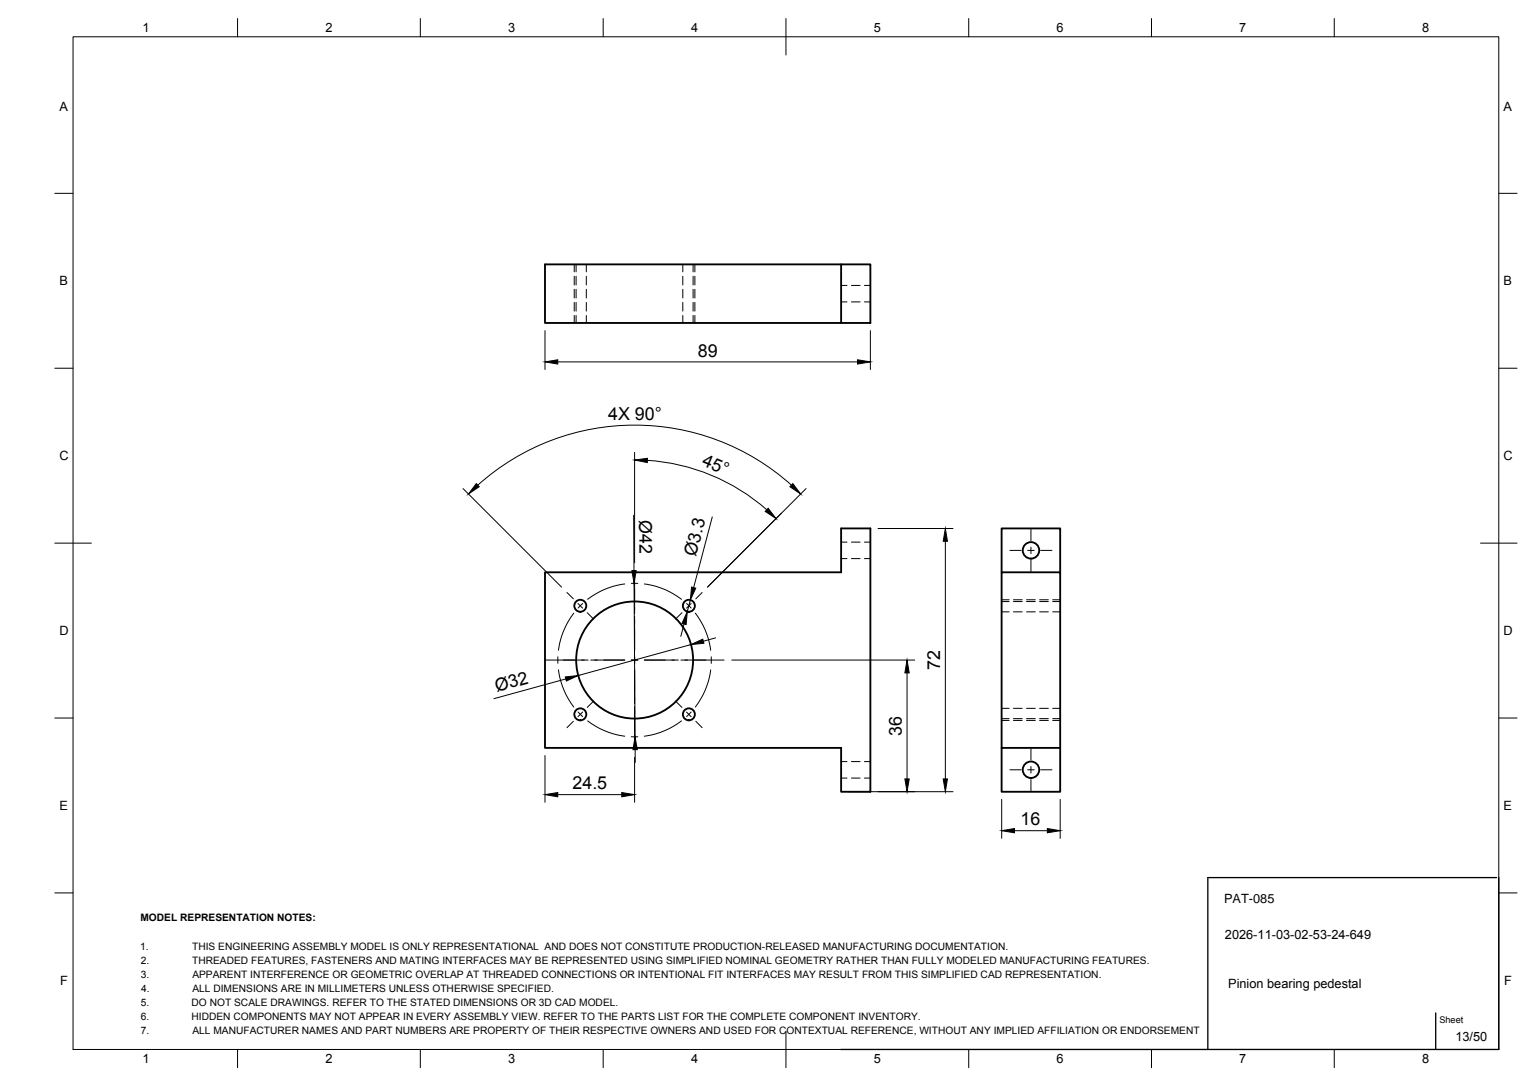
ISO-10303-21;
HEADER;
/* Generated by software containing ST-Developer
 * from STEP Tools, Inc. (www.steptools.com) 
 */

FILE_DESCRIPTION(
/* description */ ('Rack and pinion manual slide'),
/* implementation_level */ '2;1');

FILE_NAME(
/* name */ 'Pinion bearing pedestal.step',
/* time_stamp */ '2026-10-28T03:22:49-07:00',
/* author */ (''),
/* organization */ (''),
/* preprocessor_version */ 'ST-DEVELOPER v20.2',
/* originating_system */ 'Autodesk Translation Framework v15.17.0.0',
/* authorisation */ '');

FILE_SCHEMA (('AUTOMOTIVE_DESIGN { 1 0 10303 214 3 1 1 }'));
ENDSEC;

DATA;
#10=MECHANICAL_DESIGN_GEOMETRIC_PRESENTATION_REPRESENTATION('',(#740),#34851);
#648=SHAPE_REPRESENTATION_RELATIONSHIP('SRR','None',#35083,#694);
#694=ADVANCED_BREP_SHAPE_REPRESENTATION('',(#793),#34808);
#740=STYLED_ITEM('',(#35411),#793);
#793=MANIFOLD_SOLID_BREP('Body1',#13760);
#885=FACE_BOUND('',#2414,.T.);
#886=FACE_BOUND('',#2416,.T.);
#887=FACE_BOUND('',#2420,.T.);
#888=FACE_BOUND('',#2421,.T.);
#889=FACE_BOUND('',#2422,.T.);
#890=FACE_BOUND('',#2423,.T.);
#891=FACE_BOUND('',#2424,.T.);
#892=FACE_BOUND('',#2427,.T.);
#893=FACE_BOUND('',#2428,.T.);
#894=FACE_BOUND('',#2429,.T.);
#895=FACE_BOUND('',#2430,.T.);
#896=FACE_BOUND('',#2431,.T.);
#897=FACE_BOUND('',#2435,.T.);
#898=FACE_BOUND('',#2436,.T.);
#1096=PLANE('',#14485);
#1097=PLANE('',#14486);
#1098=PLANE('',#14487);
#1099=PLANE('',#14488);
#1100=PLANE('',#14489);
#1101=PLANE('',#14490);
#1102=PLANE('',#14491);
#1103=PLANE('',#14492);
#1104=PLANE('',#14493);
#1105=PLANE('',#14494);
#1615=FACE_OUTER_BOUND('',#2406,.T.);
#1616=FACE_OUTER_BOUND('',#2407,.T.);
#1617=FACE_OUTER_BOUND('',#2408,.T.);
#1618=FACE_OUTER_BOUND('',#2409,.T.);
#1619=FACE_OUTER_BOUND('',#2410,.T.);
#1620=FACE_OUTER_BOUND('',#2411,.T.);
#1621=FACE_OUTER_BOUND('',#2412,.T.);
#1622=FACE_OUTER_BOUND('',#2413,.T.);
#1623=FACE_OUTER_BOUND('',#2415,.T.);
#1624=FACE_OUTER_BOUND('',#2417,.T.);
#1625=FACE_OUTER_BOUND('',#2418,.T.);
#1626=FACE_OUTER_BOUND('',#2419,.T.);
#1627=FACE_OUTER_BOUND('',#2425,.T.);
#1628=FACE_OUTER_BOUND('',#2426,.T.);
#1629=FACE_OUTER_BOUND('',#2432,.T.);
#1630=FACE_OUTER_BOUND('',#2433,.T.);
#1631=FACE_OUTER_BOUND('',#2434,.T.);
#2406=EDGE_LOOP('',(#9594,#9595,#9596,#9597));
#2407=EDGE_LOOP('',(#9598,#9599,#9600,#9601));
#2408=EDGE_LOOP('',(#9602,#9603,#9604,#9605));
#2409=EDGE_LOOP('',(#9606,#9607,#9608,#9609));
#2410=EDGE_LOOP('',(#9610,#9611,#9612,#9613));
#2411=EDGE_LOOP('',(#9614,#9615,#9616,#9617));
#2412=EDGE_LOOP('',(#9618,#9619,#9620,#9621));
#2413=EDGE_LOOP('',(#9622,#9623,#9624,#9625));
#2414=EDGE_LOOP('',(#9626));
#2415=EDGE_LOOP('',(#9627,#9628,#9629,#9630));
#2416=EDGE_LOOP('',(#9631));
#2417=EDGE_LOOP('',(#9632,#9633,#9634,#9635));
#2418=EDGE_LOOP('',(#9636,#9637,#9638,#9639));
#2419=EDGE_LOOP('',(#9640,#9641,#9642,#9643,#9644,#9645,#9646,#9647));
#2420=EDGE_LOOP('',(#9648));
#2421=EDGE_LOOP('',(#9649));
#2422=EDGE_LOOP('',(#9650));
#2423=EDGE_LOOP('',(#9651));
#2424=EDGE_LOOP('',(#9652));
#2425=EDGE_LOOP('',(#9653,#9654,#9655,#9656));
#2426=EDGE_LOOP('',(#9657,#9658,#9659,#9660,#9661,#9662,#9663,#9664));
#2427=EDGE_LOOP('',(#9665));
#2428=EDGE_LOOP('',(#9666));
#2429=EDGE_LOOP('',(#9667));
#2430=EDGE_LOOP('',(#9668));
#2431=EDGE_LOOP('',(#9669));
#2432=EDGE_LOOP('',(#9670,#9671,#9672,#9673));
#2433=EDGE_LOOP('',(#9674,#9675,#9676,#9677));
#2434=EDGE_LOOP('',(#9678,#9679,#9680,#9681));
#2435=EDGE_LOOP('',(#9682));
#2436=EDGE_LOOP('',(#9683));
#3348=LINE('',#19852,#4639);
#3349=LINE('',#19858,#4640);
#3350=LINE('',#19864,#4641);
#3351=LINE('',#19870,#4642);
#3352=LINE('',#19876,#4643);
#3353=LINE('',#19882,#4644);
#3354=LINE('',#19888,#4645);
#3355=LINE('',#19893,#4646);
#3356=LINE('',#19895,#4647);
#3357=LINE('',#19897,#4648);
#3358=LINE('',#19898,#4649);
#3359=LINE('',#19902,#4650);
#3360=LINE('',#19904,#4651);
#3361=LINE('',#19906,#4652);
#3362=LINE('',#19907,#4653);
#3363=LINE('',#19910,#4654);
#3364=LINE('',#19912,#4655);
#3365=LINE('',#19913,#4656);
#3366=LINE('',#19916,#4657);
#3367=LINE('',#19918,#4658);
#3368=LINE('',#19919,#4659);
#3369=LINE('',#19922,#4660);
#3370=LINE('',#19924,#4661);
#3371=LINE('',#19925,#4662);
#3372=LINE('',#19926,#4663);
#3373=LINE('',#19929,#4664);
#3374=LINE('',#19930,#4665);
#3375=LINE('',#19933,#4666);
#3376=LINE('',#19934,#4667);
#3377=LINE('',#19935,#4668);
#3378=LINE('',#19937,#4669);
#4639=VECTOR('',#16022,0.225);
#4640=VECTOR('',#16029,0.225);
#4641=VECTOR('',#16036,0.164999999999999);
#4642=VECTOR('',#16043,0.164999999999999);
#4643=VECTOR('',#16050,0.164999999999999);
#4644=VECTOR('',#16057,0.164999999999999);
#4645=VECTOR('',#16064,1.6);
#4646=VECTOR('',#16069,1.);
#4647=VECTOR('',#16070,1.);
#4648=VECTOR('',#16071,1.);
#4649=VECTOR('',#16072,1.);
#4650=VECTOR('',#16075,1.);
#4651=VECTOR('',#16076,1.);
#4652=VECTOR('',#16077,1.);
#4653=VECTOR('',#16078,1.);
#4654=VECTOR('',#16081,1.);
#4655=VECTOR('',#16082,1.);
#4656=VECTOR('',#16083,1.);
#4657=VECTOR('',#16086,1.);
#4658=VECTOR('',#16087,1.);
#4659=VECTOR('',#16088,1.);
#4660=VECTOR('',#16091,1.);
#4661=VECTOR('',#16092,1.);
#4662=VECTOR('',#16093,1.);
#4663=VECTOR('',#16094,1.);
#4664=VECTOR('',#16097,1.);
#4665=VECTOR('',#16098,1.);
#4666=VECTOR('',#16101,1.);
#4667=VECTOR('',#16102,1.);
#4668=VECTOR('',#16103,1.);
#4669=VECTOR('',#16106,1.);
#5862=CIRCLE('',#14465,0.225);
#5863=CIRCLE('',#14466,0.225);
#5864=CIRCLE('',#14468,0.225);
#5865=CIRCLE('',#14469,0.225);
#5866=CIRCLE('',#14471,0.164999999999999);
#5867=CIRCLE('',#14472,0.164999999999999);
#5868=CIRCLE('',#14474,0.164999999999999);
#5869=CIRCLE('',#14475,0.164999999999999);
#5870=CIRCLE('',#14477,0.164999999999999);
#5871=CIRCLE('',#14478,0.164999999999999);
#5872=CIRCLE('',#14480,0.164999999999999);
#5873=CIRCLE('',#14481,0.164999999999999);
#5874=CIRCLE('',#14483,1.6);
#5875=CIRCLE('',#14484,1.6);
#6344=VERTEX_POINT('',#19849);
#6345=VERTEX_POINT('',#19851);
#6346=VERTEX_POINT('',#19855);
#6347=VERTEX_POINT('',#19857);
#6348=VERTEX_POINT('',#19861);
#6349=VERTEX_POINT('',#19863);
#6350=VERTEX_POINT('',#19867);
#6351=VERTEX_POINT('',#19869);
#6352=VERTEX_POINT('',#19873);
#6353=VERTEX_POINT('',#19875);
#6354=VERTEX_POINT('',#19879);
#6355=VERTEX_POINT('',#19881);
#6356=VERTEX_POINT('',#19885);
#6357=VERTEX_POINT('',#19887);
#6358=VERTEX_POINT('',#19891);
#6359=VERTEX_POINT('',#19892);
#6360=VERTEX_POINT('',#19894);
#6361=VERTEX_POINT('',#19896);
#6362=VERTEX_POINT('',#19900);
#6363=VERTEX_POINT('',#19901);
#6364=VERTEX_POINT('',#19903);
#6365=VERTEX_POINT('',#19905);
#6366=VERTEX_POINT('',#19909);
#6367=VERTEX_POINT('',#19911);
#6368=VERTEX_POINT('',#19915);
#6369=VERTEX_POINT('',#19917);
#6370=VERTEX_POINT('',#19921);
#6371=VERTEX_POINT('',#19923);
#6372=VERTEX_POINT('',#19928);
#6373=VERTEX_POINT('',#19932);
#7609=EDGE_CURVE('',#6344,#6344,#5862,.T.);
#7610=EDGE_CURVE('',#6344,#6345,#3348,.T.);
#7611=EDGE_CURVE('',#6345,#6345,#5863,.T.);
#7612=EDGE_CURVE('',#6346,#6346,#5864,.T.);
#7613=EDGE_CURVE('',#6346,#6347,#3349,.T.);
#7614=EDGE_CURVE('',#6347,#6347,#5865,.T.);
#7615=EDGE_CURVE('',#6348,#6348,#5866,.T.);
#7616=EDGE_CURVE('',#6348,#6349,#3350,.T.);
#7617=EDGE_CURVE('',#6349,#6349,#5867,.T.);
#7618=EDGE_CURVE('',#6350,#6350,#5868,.T.);
#7619=EDGE_CURVE('',#6350,#6351,#3351,.T.);
#7620=EDGE_CURVE('',#6351,#6351,#5869,.T.);
#7621=EDGE_CURVE('',#6352,#6352,#5870,.T.);
#7622=EDGE_CURVE('',#6352,#6353,#3352,.T.);
#7623=EDGE_CURVE('',#6353,#6353,#5871,.T.);
#7624=EDGE_CURVE('',#6354,#6354,#5872,.T.);
#7625=EDGE_CURVE('',#6354,#6355,#3353,.T.);
#7626=EDGE_CURVE('',#6355,#6355,#5873,.T.);
#7627=EDGE_CURVE('',#6356,#6356,#5874,.T.);
#7628=EDGE_CURVE('',#6356,#6357,#3354,.T.);
#7629=EDGE_CURVE('',#6357,#6357,#5875,.T.);
#7630=EDGE_CURVE('',#6358,#6359,#3355,.T.);
#7631=EDGE_CURVE('',#6360,#6358,#3356,.T.);
#7632=EDGE_CURVE('',#6360,#6361,#3357,.T.);
#7633=EDGE_CURVE('',#6359,#6361,#3358,.T.);
#7634=EDGE_CURVE('',#6362,#6363,#3359,.T.);
#7635=EDGE_CURVE('',#6364,#6362,#3360,.T.);
#7636=EDGE_CURVE('',#6365,#6364,#3361,.T.);
#7637=EDGE_CURVE('',#6363,#6365,#3362,.T.);
#7638=EDGE_CURVE('',#6365,#6366,#3363,.T.);
#7639=EDGE_CURVE('',#6367,#6364,#3364,.T.);
#7640=EDGE_CURVE('',#6366,#6367,#3365,.T.);
#7641=EDGE_CURVE('',#6368,#6360,#3366,.T.);
#7642=EDGE_CURVE('',#6368,#6369,#3367,.T.);
#7643=EDGE_CURVE('',#6361,#6369,#3368,.T.);
#7644=EDGE_CURVE('',#6358,#6370,#3369,.T.);
#7645=EDGE_CURVE('',#6371,#6370,#3370,.T.);
#7646=EDGE_CURVE('',#6363,#6371,#3371,.T.);
#7647=EDGE_CURVE('',#6366,#6368,#3372,.T.);
#7648=EDGE_CURVE('',#6359,#6372,#3373,.T.);
#7649=EDGE_CURVE('',#6370,#6372,#3374,.T.);
#7650=EDGE_CURVE('',#6362,#6373,#3375,.T.);
#7651=EDGE_CURVE('',#6372,#6373,#3376,.T.);
#7652=EDGE_CURVE('',#6369,#6367,#3377,.T.);
#7653=EDGE_CURVE('',#6373,#6371,#3378,.T.);
#9594=ORIENTED_EDGE('',*,*,#7609,.F.);
#9595=ORIENTED_EDGE('',*,*,#7610,.T.);
#9596=ORIENTED_EDGE('',*,*,#7611,.F.);
#9597=ORIENTED_EDGE('',*,*,#7610,.F.);
#9598=ORIENTED_EDGE('',*,*,#7612,.F.);
#9599=ORIENTED_EDGE('',*,*,#7613,.T.);
#9600=ORIENTED_EDGE('',*,*,#7614,.F.);
#9601=ORIENTED_EDGE('',*,*,#7613,.F.);
#9602=ORIENTED_EDGE('',*,*,#7615,.F.);
#9603=ORIENTED_EDGE('',*,*,#7616,.T.);
#9604=ORIENTED_EDGE('',*,*,#7617,.F.);
#9605=ORIENTED_EDGE('',*,*,#7616,.F.);
#9606=ORIENTED_EDGE('',*,*,#7618,.F.);
#9607=ORIENTED_EDGE('',*,*,#7619,.T.);
#9608=ORIENTED_EDGE('',*,*,#7620,.F.);
#9609=ORIENTED_EDGE('',*,*,#7619,.F.);
#9610=ORIENTED_EDGE('',*,*,#7621,.F.);
#9611=ORIENTED_EDGE('',*,*,#7622,.T.);
#9612=ORIENTED_EDGE('',*,*,#7623,.F.);
#9613=ORIENTED_EDGE('',*,*,#7622,.F.);
#9614=ORIENTED_EDGE('',*,*,#7624,.F.);
#9615=ORIENTED_EDGE('',*,*,#7625,.T.);
#9616=ORIENTED_EDGE('',*,*,#7626,.F.);
#9617=ORIENTED_EDGE('',*,*,#7625,.F.);
#9618=ORIENTED_EDGE('',*,*,#7627,.F.);
#9619=ORIENTED_EDGE('',*,*,#7628,.T.);
#9620=ORIENTED_EDGE('',*,*,#7629,.F.);
#9621=ORIENTED_EDGE('',*,*,#7628,.F.);
#9622=ORIENTED_EDGE('',*,*,#7630,.F.);
#9623=ORIENTED_EDGE('',*,*,#7631,.F.);
#9624=ORIENTED_EDGE('',*,*,#7632,.T.);
#9625=ORIENTED_EDGE('',*,*,#7633,.F.);
#9626=ORIENTED_EDGE('',*,*,#7614,.T.);
#9627=ORIENTED_EDGE('',*,*,#7634,.F.);
#9628=ORIENTED_EDGE('',*,*,#7635,.F.);
#9629=ORIENTED_EDGE('',*,*,#7636,.F.);
#9630=ORIENTED_EDGE('',*,*,#7637,.F.);
#9631=ORIENTED_EDGE('',*,*,#7611,.T.);
#9632=ORIENTED_EDGE('',*,*,#7638,.F.);
#9633=ORIENTED_EDGE('',*,*,#7636,.T.);
#9634=ORIENTED_EDGE('',*,*,#7639,.F.);
#9635=ORIENTED_EDGE('',*,*,#7640,.F.);
#9636=ORIENTED_EDGE('',*,*,#7641,.F.);
#9637=ORIENTED_EDGE('',*,*,#7642,.T.);
#9638=ORIENTED_EDGE('',*,*,#7643,.F.);
#9639=ORIENTED_EDGE('',*,*,#7632,.F.);
#9640=ORIENTED_EDGE('',*,*,#7644,.T.);
#9641=ORIENTED_EDGE('',*,*,#7645,.F.);
#9642=ORIENTED_EDGE('',*,*,#7646,.F.);
#9643=ORIENTED_EDGE('',*,*,#7637,.T.);
#9644=ORIENTED_EDGE('',*,*,#7638,.T.);
#9645=ORIENTED_EDGE('',*,*,#7647,.T.);
#9646=ORIENTED_EDGE('',*,*,#7641,.T.);
#9647=ORIENTED_EDGE('',*,*,#7631,.T.);
#9648=ORIENTED_EDGE('',*,*,#7627,.T.);
#9649=ORIENTED_EDGE('',*,*,#7624,.T.);
#9650=ORIENTED_EDGE('',*,*,#7621,.T.);
#9651=ORIENTED_EDGE('',*,*,#7618,.T.);
#9652=ORIENTED_EDGE('',*,*,#7615,.T.);
#9653=ORIENTED_EDGE('',*,*,#7630,.T.);
#9654=ORIENTED_EDGE('',*,*,#7648,.T.);
#9655=ORIENTED_EDGE('',*,*,#7649,.F.);
#9656=ORIENTED_EDGE('',*,*,#7644,.F.);
#9657=ORIENTED_EDGE('',*,*,#7650,.T.);
#9658=ORIENTED_EDGE('',*,*,#7651,.F.);
#9659=ORIENTED_EDGE('',*,*,#7648,.F.);
#9660=ORIENTED_EDGE('',*,*,#7633,.T.);
#9661=ORIENTED_EDGE('',*,*,#7643,.T.);
#9662=ORIENTED_EDGE('',*,*,#7652,.T.);
#9663=ORIENTED_EDGE('',*,*,#7639,.T.);
#9664=ORIENTED_EDGE('',*,*,#7635,.T.);
#9665=ORIENTED_EDGE('',*,*,#7629,.T.);
#9666=ORIENTED_EDGE('',*,*,#7626,.T.);
#9667=ORIENTED_EDGE('',*,*,#7623,.T.);
#9668=ORIENTED_EDGE('',*,*,#7620,.T.);
#9669=ORIENTED_EDGE('',*,*,#7617,.T.);
#9670=ORIENTED_EDGE('',*,*,#7634,.T.);
#9671=ORIENTED_EDGE('',*,*,#7646,.T.);
#9672=ORIENTED_EDGE('',*,*,#7653,.F.);
#9673=ORIENTED_EDGE('',*,*,#7650,.F.);
#9674=ORIENTED_EDGE('',*,*,#7653,.T.);
#9675=ORIENTED_EDGE('',*,*,#7645,.T.);
#9676=ORIENTED_EDGE('',*,*,#7649,.T.);
#9677=ORIENTED_EDGE('',*,*,#7651,.T.);
#9678=ORIENTED_EDGE('',*,*,#7652,.F.);
#9679=ORIENTED_EDGE('',*,*,#7642,.F.);
#9680=ORIENTED_EDGE('',*,*,#7647,.F.);
#9681=ORIENTED_EDGE('',*,*,#7640,.T.);
#9682=ORIENTED_EDGE('',*,*,#7609,.T.);
#9683=ORIENTED_EDGE('',*,*,#7612,.T.);
#12872=CYLINDRICAL_SURFACE('',#14464,0.225);
#12873=CYLINDRICAL_SURFACE('',#14467,0.225);
#12874=CYLINDRICAL_SURFACE('',#14470,0.164999999999999);
#12875=CYLINDRICAL_SURFACE('',#14473,0.164999999999999);
#12876=CYLINDRICAL_SURFACE('',#14476,0.164999999999999);
#12877=CYLINDRICAL_SURFACE('',#14479,0.164999999999999);
#12878=CYLINDRICAL_SURFACE('',#14482,1.6);
#13093=ADVANCED_FACE('',(#1615),#12872,.F.);
#13094=ADVANCED_FACE('',(#1616),#12873,.F.);
#13095=ADVANCED_FACE('',(#1617),#12874,.F.);
#13096=ADVANCED_FACE('',(#1618),#12875,.F.);
#13097=ADVANCED_FACE('',(#1619),#12876,.F.);
#13098=ADVANCED_FACE('',(#1620),#12877,.F.);
#13099=ADVANCED_FACE('',(#1621),#12878,.F.);
#13100=ADVANCED_FACE('',(#1622,#885),#1096,.T.);
#13101=ADVANCED_FACE('',(#1623,#886),#1097,.T.);
#13102=ADVANCED_FACE('',(#1624),#1098,.T.);
#13103=ADVANCED_FACE('',(#1625),#1099,.T.);
#13104=ADVANCED_FACE('',(#1626,#887,#888,#889,#890,#891),#1100,.T.);
#13105=ADVANCED_FACE('',(#1627),#1101,.T.);
#13106=ADVANCED_FACE('',(#1628,#892,#893,#894,#895,#896),#1102,.T.);
#13107=ADVANCED_FACE('',(#1629),#1103,.T.);
#13108=ADVANCED_FACE('',(#1630),#1104,.T.);
#13109=ADVANCED_FACE('',(#1631,#897,#898),#1105,.F.);
#13760=CLOSED_SHELL('',(#13093,#13094,#13095,#13096,#13097,#13098,#13099,
#13100,#13101,#13102,#13103,#13104,#13105,#13106,#13107,#13108,#13109));
#14463=AXIS2_PLACEMENT_3D('',#19847,#16016,#16017);
#14464=AXIS2_PLACEMENT_3D('',#19848,#16018,#16019);
#14465=AXIS2_PLACEMENT_3D('',#19850,#16020,#16021);
#14466=AXIS2_PLACEMENT_3D('',#19853,#16023,#16024);
#14467=AXIS2_PLACEMENT_3D('',#19854,#16025,#16026);
#14468=AXIS2_PLACEMENT_3D('',#19856,#16027,#16028);
#14469=AXIS2_PLACEMENT_3D('',#19859,#16030,#16031);
#14470=AXIS2_PLACEMENT_3D('',#19860,#16032,#16033);
#14471=AXIS2_PLACEMENT_3D('',#19862,#16034,#16035);
#14472=AXIS2_PLACEMENT_3D('',#19865,#16037,#16038);
#14473=AXIS2_PLACEMENT_3D('',#19866,#16039,#16040);
#14474=AXIS2_PLACEMENT_3D('',#19868,#16041,#16042);
#14475=AXIS2_PLACEMENT_3D('',#19871,#16044,#16045);
#14476=AXIS2_PLACEMENT_3D('',#19872,#16046,#16047);
#14477=AXIS2_PLACEMENT_3D('',#19874,#16048,#16049);
#14478=AXIS2_PLACEMENT_3D('',#19877,#16051,#16052);
#14479=AXIS2_PLACEMENT_3D('',#19878,#16053,#16054);
#14480=AXIS2_PLACEMENT_3D('',#19880,#16055,#16056);
#14481=AXIS2_PLACEMENT_3D('',#19883,#16058,#16059);
#14482=AXIS2_PLACEMENT_3D('',#19884,#16060,#16061);
#14483=AXIS2_PLACEMENT_3D('',#19886,#16062,#16063);
#14484=AXIS2_PLACEMENT_3D('',#19889,#16065,#16066);
#14485=AXIS2_PLACEMENT_3D('',#19890,#16067,#16068);
#14486=AXIS2_PLACEMENT_3D('',#19899,#16073,#16074);
#14487=AXIS2_PLACEMENT_3D('',#19908,#16079,#16080);
#14488=AXIS2_PLACEMENT_3D('',#19914,#16084,#16085);
#14489=AXIS2_PLACEMENT_3D('',#19920,#16089,#16090);
#14490=AXIS2_PLACEMENT_3D('',#19927,#16095,#16096);
#14491=AXIS2_PLACEMENT_3D('',#19931,#16099,#16100);
#14492=AXIS2_PLACEMENT_3D('',#19936,#16104,#16105);
#14493=AXIS2_PLACEMENT_3D('',#19938,#16107,#16108);
#14494=AXIS2_PLACEMENT_3D('',#19939,#16109,#16110);
#16016=DIRECTION('axis',(0.,0.,1.));
#16017=DIRECTION('refdir',(1.,0.,0.));
#16018=DIRECTION('center_axis',(0.,0.,1.));
#16019=DIRECTION('ref_axis',(1.,0.,0.));
#16020=DIRECTION('center_axis',(0.,0.,1.));
#16021=DIRECTION('ref_axis',(1.,0.,0.));
#16022=DIRECTION('',(0.,0.,1.));
#16023=DIRECTION('center_axis',(0.,0.,-1.));
#16024=DIRECTION('ref_axis',(1.,0.,0.));
#16025=DIRECTION('center_axis',(0.,0.,1.));
#16026=DIRECTION('ref_axis',(1.,0.,0.));
#16027=DIRECTION('center_axis',(0.,0.,1.));
#16028=DIRECTION('ref_axis',(1.,0.,0.));
#16029=DIRECTION('',(0.,0.,1.));
#16030=DIRECTION('center_axis',(0.,0.,-1.));
#16031=DIRECTION('ref_axis',(1.,0.,0.));
#16032=DIRECTION('center_axis',(0.,1.,0.));
#16033=DIRECTION('ref_axis',(1.,0.,0.));
#16034=DIRECTION('center_axis',(0.,1.,0.));
#16035=DIRECTION('ref_axis',(1.,0.,0.));
#16036=DIRECTION('',(0.,1.,0.));
#16037=DIRECTION('center_axis',(0.,-1.,0.));
#16038=DIRECTION('ref_axis',(1.,0.,0.));
#16039=DIRECTION('center_axis',(0.,1.,0.));
#16040=DIRECTION('ref_axis',(1.,0.,0.));
#16041=DIRECTION('center_axis',(0.,1.,0.));
#16042=DIRECTION('ref_axis',(1.,0.,0.));
#16043=DIRECTION('',(0.,1.,0.));
#16044=DIRECTION('center_axis',(0.,-1.,0.));
#16045=DIRECTION('ref_axis',(1.,0.,0.));
#16046=DIRECTION('center_axis',(0.,1.,0.));
#16047=DIRECTION('ref_axis',(1.,0.,0.));
#16048=DIRECTION('center_axis',(0.,1.,0.));
#16049=DIRECTION('ref_axis',(1.,0.,0.));
#16050=DIRECTION('',(0.,1.,0.));
#16051=DIRECTION('center_axis',(0.,-1.,0.));
#16052=DIRECTION('ref_axis',(1.,0.,0.));
#16053=DIRECTION('center_axis',(0.,1.,0.));
#16054=DIRECTION('ref_axis',(1.,0.,0.));
#16055=DIRECTION('center_axis',(0.,1.,0.));
#16056=DIRECTION('ref_axis',(1.,0.,0.));
#16057=DIRECTION('',(0.,1.,0.));
#16058=DIRECTION('center_axis',(0.,-1.,0.));
#16059=DIRECTION('ref_axis',(1.,0.,0.));
#16060=DIRECTION('center_axis',(0.,1.,0.));
#16061=DIRECTION('ref_axis',(1.,0.,0.));
#16062=DIRECTION('center_axis',(0.,1.,0.));
#16063=DIRECTION('ref_axis',(1.,0.,0.));
#16064=DIRECTION('',(0.,1.,0.));
#16065=DIRECTION('center_axis',(0.,-1.,0.));
#16066=DIRECTION('ref_axis',(1.,0.,0.));
#16067=DIRECTION('center_axis',(0.,0.,1.));
#16068=DIRECTION('ref_axis',(1.,0.,0.));
#16069=DIRECTION('',(0.,1.,0.));
#16070=DIRECTION('',(-1.,0.,0.));
#16071=DIRECTION('',(0.,1.,0.));
#16072=DIRECTION('',(1.,0.,0.));
#16073=DIRECTION('center_axis',(0.,0.,1.));
#16074=DIRECTION('ref_axis',(1.,0.,0.));
#16075=DIRECTION('',(0.,-1.,0.));
#16076=DIRECTION('',(1.,0.,0.));
#16077=DIRECTION('',(0.,1.,0.));
#16078=DIRECTION('',(-1.,0.,0.));
#16079=DIRECTION('center_axis',(-1.,0.,0.));
#16080=DIRECTION('ref_axis',(0.,0.,1.));
#16081=DIRECTION('',(0.,0.,-1.));
#16082=DIRECTION('',(0.,0.,1.));
#16083=DIRECTION('',(0.,1.,0.));
#16084=DIRECTION('center_axis',(1.,0.,0.));
#16085=DIRECTION('ref_axis',(0.,0.,-1.));
#16086=DIRECTION('',(0.,0.,1.));
#16087=DIRECTION('',(0.,1.,0.));
#16088=DIRECTION('',(0.,0.,-1.));
#16089=DIRECTION('center_axis',(0.,-1.,0.));
#16090=DIRECTION('ref_axis',(1.,0.,0.));
#16091=DIRECTION('',(0.,0.,1.));
#16092=DIRECTION('',(1.,0.,0.));
#16093=DIRECTION('',(0.,0.,1.));
#16094=DIRECTION('',(1.,0.,0.));
#16095=DIRECTION('center_axis',(1.,0.,0.));
#16096=DIRECTION('ref_axis',(0.,1.,0.));
#16097=DIRECTION('',(0.,0.,1.));
#16098=DIRECTION('',(0.,1.,0.));
#16099=DIRECTION('center_axis',(0.,1.,0.));
#16100=DIRECTION('ref_axis',(-1.,0.,0.));
#16101=DIRECTION('',(0.,0.,1.));
#16102=DIRECTION('',(-1.,0.,0.));
#16103=DIRECTION('',(-1.,0.,0.));
#16104=DIRECTION('center_axis',(-1.,0.,0.));
#16105=DIRECTION('ref_axis',(0.,-1.,0.));
#16106=DIRECTION('',(0.,-1.,0.));
#16107=DIRECTION('center_axis',(0.,0.,1.));
#16108=DIRECTION('ref_axis',(1.,0.,0.));
#16109=DIRECTION('center_axis',(0.,0.,1.));
#16110=DIRECTION('ref_axis',(1.,0.,0.));
#19847=CARTESIAN_POINT('',(0.,0.,0.));
#19848=CARTESIAN_POINT('Origin',(8.,-4.2,3.7));
#19849=CARTESIAN_POINT('',(7.775,-4.2,3.8));
#19850=CARTESIAN_POINT('Origin',(8.,-4.2,3.8));
#19851=CARTESIAN_POINT('',(7.775,-4.2,4.6));
#19852=CARTESIAN_POINT('',(7.775,-4.2,3.7));
#19853=CARTESIAN_POINT('Origin',(8.,-4.2,4.6));
#19854=CARTESIAN_POINT('Origin',(14.,-4.2,3.7));
#19855=CARTESIAN_POINT('',(13.775,-4.2,3.8));
#19856=CARTESIAN_POINT('Origin',(14.,-4.2,3.8));
#19857=CARTESIAN_POINT('',(13.775,-4.2,4.6));
#19858=CARTESIAN_POINT('',(13.775,-4.2,3.7));
#19859=CARTESIAN_POINT('Origin',(14.,-4.2,4.6));
#19860=CARTESIAN_POINT('Origin',(9.51507575950825,-5.1,8.76507575950825));
#19861=CARTESIAN_POINT('',(9.35007575950825,-5.,8.76507575950825));
#19862=CARTESIAN_POINT('Origin',(9.51507575950825,-5.,8.76507575950825));
#19863=CARTESIAN_POINT('',(9.35007575950825,-3.4,8.76507575950825));
#19864=CARTESIAN_POINT('',(9.35007575950825,-5.1,8.76507575950825));
#19865=CARTESIAN_POINT('Origin',(9.51507575950825,-3.4,8.76507575950825));
#19866=CARTESIAN_POINT('Origin',(9.51507575950825,-5.1,11.7349242404918));
#19867=CARTESIAN_POINT('',(9.35007575950825,-5.,11.7349242404918));
#19868=CARTESIAN_POINT('Origin',(9.51507575950825,-5.,11.7349242404918));
#19869=CARTESIAN_POINT('',(9.35007575950825,-3.4,11.7349242404918));
#19870=CARTESIAN_POINT('',(9.35007575950825,-5.1,11.7349242404918));
#19871=CARTESIAN_POINT('Origin',(9.51507575950825,-3.4,11.7349242404918));
#19872=CARTESIAN_POINT('Origin',(12.4849242404918,-5.1,11.7349242404918));
#19873=CARTESIAN_POINT('',(12.3199242404918,-5.,11.7349242404918));
#19874=CARTESIAN_POINT('Origin',(12.4849242404918,-5.,11.7349242404918));
#19875=CARTESIAN_POINT('',(12.3199242404918,-3.4,11.7349242404918));
#19876=CARTESIAN_POINT('',(12.3199242404918,-5.1,11.7349242404918));
#19877=CARTESIAN_POINT('Origin',(12.4849242404918,-3.4,11.7349242404918));
#19878=CARTESIAN_POINT('Origin',(12.4849242404917,-5.1,8.76507575950825));
#19879=CARTESIAN_POINT('',(12.3199242404917,-5.,8.76507575950825));
#19880=CARTESIAN_POINT('Origin',(12.4849242404917,-5.,8.76507575950825));
#19881=CARTESIAN_POINT('',(12.3199242404917,-3.4,8.76507575950825));
#19882=CARTESIAN_POINT('',(12.3199242404917,-5.1,8.76507575950825));
#19883=CARTESIAN_POINT('Origin',(12.4849242404917,-3.4,8.76507575950825));
#19884=CARTESIAN_POINT('Origin',(11.,-5.1,10.25));
#19885=CARTESIAN_POINT('',(9.4,-5.,10.25));
#19886=CARTESIAN_POINT('Origin',(11.,-5.,10.25));
#19887=CARTESIAN_POINT('',(9.4,-3.4,10.25));
#19888=CARTESIAN_POINT('',(9.4,-5.1,10.25));
#19889=CARTESIAN_POINT('Origin',(11.,-3.4,10.25));
#19890=CARTESIAN_POINT('Origin',(7.4,-5.,4.6));
#19891=CARTESIAN_POINT('',(13.4,-5.,4.6));
#19892=CARTESIAN_POINT('',(13.4,-3.4,4.6));
#19893=CARTESIAN_POINT('',(13.4,-5.,4.6));
#19894=CARTESIAN_POINT('',(14.6,-5.,4.6));
#19895=CARTESIAN_POINT('',(14.6,-5.,4.6));
#19896=CARTESIAN_POINT('',(14.6,-3.4,4.6));
#19897=CARTESIAN_POINT('',(14.6,-5.,4.6));
#19898=CARTESIAN_POINT('',(14.6,-3.4,4.6));
#19899=CARTESIAN_POINT('Origin',(7.4,-5.,4.6));
#19900=CARTESIAN_POINT('',(8.6,-3.4,4.6));
#19901=CARTESIAN_POINT('',(8.6,-5.,4.6));
#19902=CARTESIAN_POINT('',(8.6,-4.2,4.6));
#19903=CARTESIAN_POINT('',(7.4,-3.4,4.6));
#19904=CARTESIAN_POINT('',(14.6,-3.4,4.6));
#19905=CARTESIAN_POINT('',(7.4,-5.,4.6));
#19906=CARTESIAN_POINT('',(7.4,-5.,4.6));
#19907=CARTESIAN_POINT('',(14.6,-5.,4.6));
#19908=CARTESIAN_POINT('Origin',(7.4,-5.,3.8));
#19909=CARTESIAN_POINT('',(7.4,-5.,3.8));
#19910=CARTESIAN_POINT('',(7.4,-5.,4.6));
#19911=CARTESIAN_POINT('',(7.4,-3.4,3.8));
#19912=CARTESIAN_POINT('',(7.4,-3.4,4.6));
#19913=CARTESIAN_POINT('',(7.4,-5.,3.8));
#19914=CARTESIAN_POINT('Origin',(14.6,-5.,4.6));
#19915=CARTESIAN_POINT('',(14.6,-5.,3.8));
#19916=CARTESIAN_POINT('',(14.6,-5.,3.8));
#19917=CARTESIAN_POINT('',(14.6,-3.4,3.8));
#19918=CARTESIAN_POINT('',(14.6,-5.,3.8));
#19919=CARTESIAN_POINT('',(14.6,-3.4,3.8));
#19920=CARTESIAN_POINT('Origin',(8.6,-5.,3.8));
#19921=CARTESIAN_POINT('',(13.4,-5.,12.7));
#19922=CARTESIAN_POINT('',(13.4,-5.,3.8));
#19923=CARTESIAN_POINT('',(8.6,-5.,12.7));
#19924=CARTESIAN_POINT('',(8.6,-5.,12.7));
#19925=CARTESIAN_POINT('',(8.6,-5.,3.8));
#19926=CARTESIAN_POINT('',(7.4,-5.,3.8));
#19927=CARTESIAN_POINT('Origin',(13.4,-5.,3.8));
#19928=CARTESIAN_POINT('',(13.4,-3.4,12.7));
#19929=CARTESIAN_POINT('',(13.4,-3.4,3.8));
#19930=CARTESIAN_POINT('',(13.4,-5.,12.7));
#19931=CARTESIAN_POINT('Origin',(13.4,-3.4,3.8));
#19932=CARTESIAN_POINT('',(8.6,-3.4,12.7));
#19933=CARTESIAN_POINT('',(8.6,-3.4,3.8));
#19934=CARTESIAN_POINT('',(13.4,-3.4,12.7));
#19935=CARTESIAN_POINT('',(7.4,-3.4,3.8));
#19936=CARTESIAN_POINT('Origin',(8.6,-3.4,3.8));
#19937=CARTESIAN_POINT('',(8.6,-3.4,12.7));
#19938=CARTESIAN_POINT('Origin',(11.,-4.2,12.7));
#19939=CARTESIAN_POINT('Origin',(11.,-4.2,3.8));
#34754=UNCERTAINTY_MEASURE_WITH_UNIT(LENGTH_MEASURE(0.001),#34852,
'DISTANCE_ACCURACY_VALUE',
'Maximum model space distance between geometric entities at asserted c
onnectivities');
#34797=UNCERTAINTY_MEASURE_WITH_UNIT(LENGTH_MEASURE(0.001),#34852,
'DISTANCE_ACCURACY_VALUE',
'Maximum model space distance between geometric entities at asserted c
onnectivities');
#34808=(
GEOMETRIC_REPRESENTATION_CONTEXT(3)
GLOBAL_UNCERTAINTY_ASSIGNED_CONTEXT((#34754))
GLOBAL_UNIT_ASSIGNED_CONTEXT((#34852,#34854,#34855))
REPRESENTATION_CONTEXT('','3D')
);
#34851=(
GEOMETRIC_REPRESENTATION_CONTEXT(3)
GLOBAL_UNCERTAINTY_ASSIGNED_CONTEXT((#34797))
GLOBAL_UNIT_ASSIGNED_CONTEXT((#34852,#34854,#34855))
REPRESENTATION_CONTEXT('','3D')
);
#34852=(
LENGTH_UNIT()
NAMED_UNIT(*)
SI_UNIT(.CENTI.,.METRE.)
);
#34854=(
NAMED_UNIT(*)
PLANE_ANGLE_UNIT()
SI_UNIT($,.RADIAN.)
);
#34855=(
NAMED_UNIT(*)
SI_UNIT($,.STERADIAN.)
SOLID_ANGLE_UNIT()
);
#34866=SHAPE_DEFINITION_REPRESENTATION(#34919,#35083);
#34919=PRODUCT_DEFINITION_SHAPE('',$,#35137);
#35083=SHAPE_REPRESENTATION('',(#14463),#34808);
#35126=PRODUCT_DEFINITION_CONTEXT('part definition',#35287,'design');
#35137=PRODUCT_DEFINITION('Pinion bearing pedestal',
'Pinion bearing pedestal',#35190,#35126);
#35190=PRODUCT_DEFINITION_FORMATION('',$,#35299);
#35287=APPLICATION_CONTEXT(
'Core Data for Automotive Mechanical Design Process');
#35288=PRODUCT_CONTEXT('part definition',#35287,'mechanical');
#35299=PRODUCT('Pinion bearing pedestal','Pinion bearing pedestal',
'Pinion bearing pedestal',(#35288));
#35405=COLOUR_RGB('Grey',0.48,0.52,0.57);
#35406=FILL_AREA_STYLE_COLOUR('',#35405);
#35407=FILL_AREA_STYLE('',(#35406));
#35408=SURFACE_STYLE_FILL_AREA(#35407);
#35409=SURFACE_SIDE_STYLE('',(#35408));
#35410=SURFACE_STYLE_USAGE(.BOTH.,#35409);
#35411=PRESENTATION_STYLE_ASSIGNMENT((#35410));
ENDSEC;
END-ISO-10303-21;
